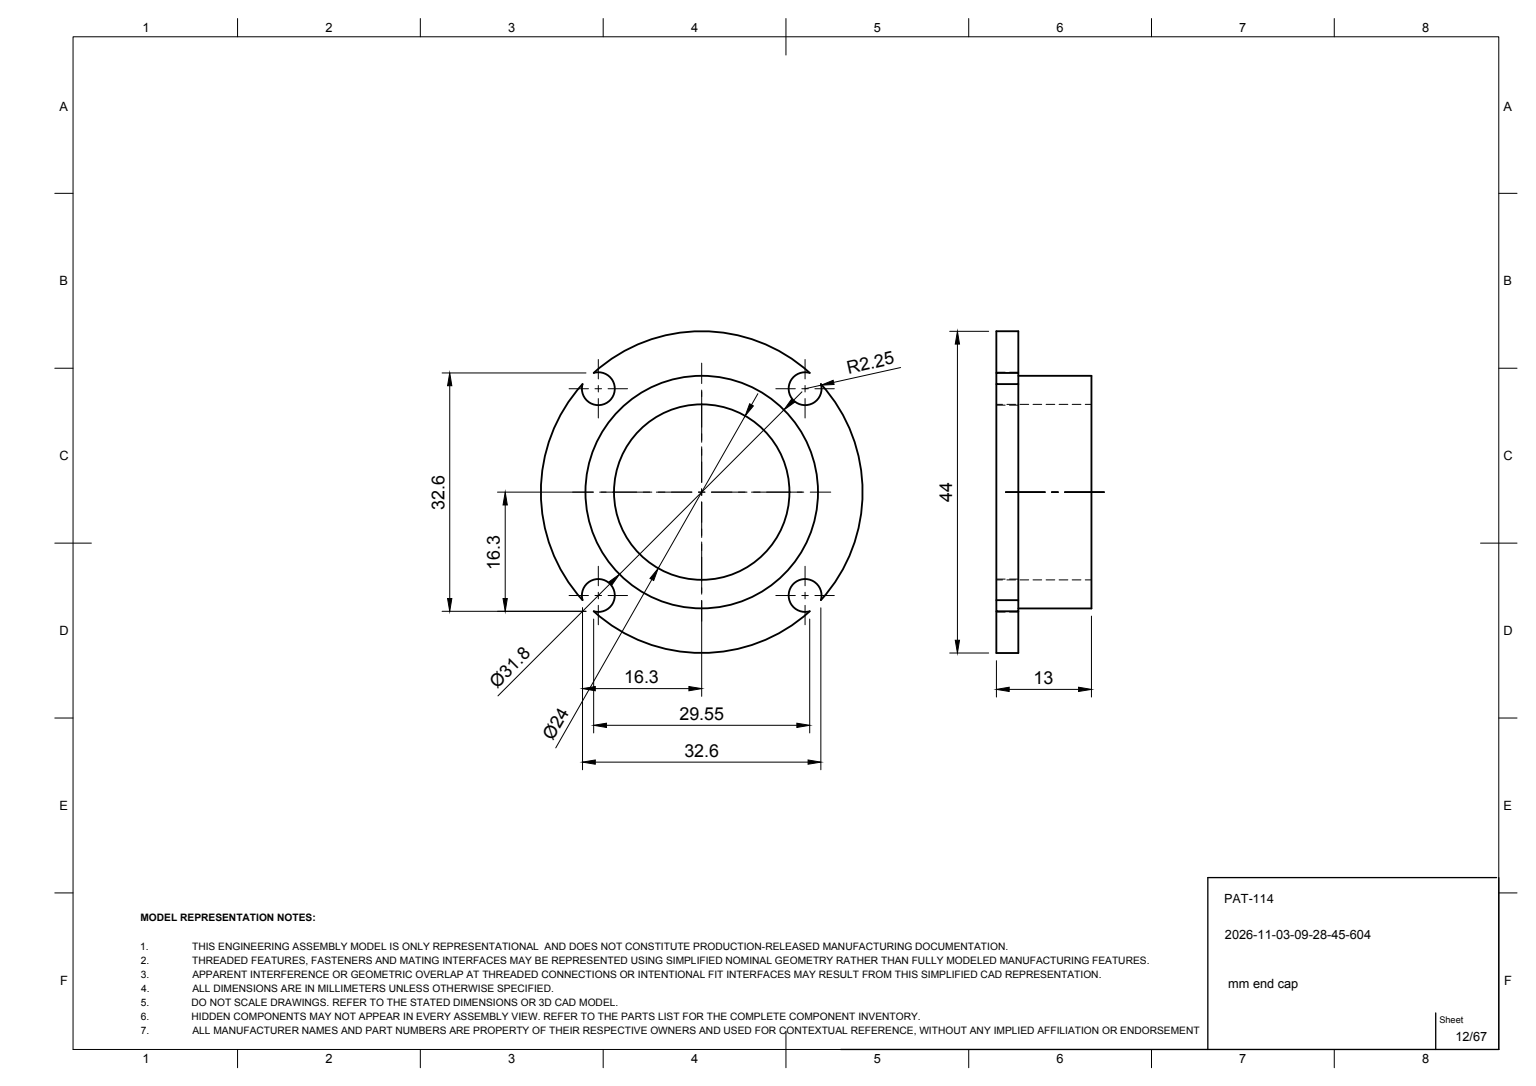
ISO-10303-21;
HEADER;
/* Generated by software containing ST-Developer
 * from STEP Tools, Inc. (www.steptools.com) 
 */

FILE_DESCRIPTION(
/* description */ ('Two-stage gear reducer in split housing'),
/* implementation_level */ '2;1');

FILE_NAME(
/* name */ 'mm end cap.step',
/* time_stamp */ '2026-10-28T03:22:31-07:00',
/* author */ (''),
/* organization */ (''),
/* preprocessor_version */ 'ST-DEVELOPER v20.2',
/* originating_system */ 'Autodesk Translation Framework v15.17.0.0',
/* authorisation */ '');

FILE_SCHEMA (('AUTOMOTIVE_DESIGN { 1 0 10303 214 3 1 1 }'));
ENDSEC;

DATA;
#10=MECHANICAL_DESIGN_GEOMETRIC_PRESENTATION_REPRESENTATION('',(#1241),#73366);
#1129=SHAPE_REPRESENTATION_RELATIONSHIP('SRR','None',#73616,#1185);
#1185=ADVANCED_BREP_SHAPE_REPRESENTATION('',(#1312),#73312);
#1241=STYLED_ITEM('',(#74002),#1312);
#1312=MANIFOLD_SOLID_BREP('Body1',#16129);
#1460=FACE_BOUND('',#3200,.T.);
#1461=FACE_BOUND('',#3207,.T.);
#1462=FACE_BOUND('',#3210,.T.);
#1708=PLANE('',#17204);
#1709=PLANE('',#17221);
#1710=PLANE('',#17224);
#2196=FACE_OUTER_BOUND('',#3195,.T.);
#2197=FACE_OUTER_BOUND('',#3196,.T.);
#2198=FACE_OUTER_BOUND('',#3197,.T.);
#2199=FACE_OUTER_BOUND('',#3198,.T.);
#2200=FACE_OUTER_BOUND('',#3199,.T.);
#2201=FACE_OUTER_BOUND('',#3201,.T.);
#2202=FACE_OUTER_BOUND('',#3202,.T.);
#2203=FACE_OUTER_BOUND('',#3203,.T.);
#2204=FACE_OUTER_BOUND('',#3204,.T.);
#2205=FACE_OUTER_BOUND('',#3205,.T.);
#2206=FACE_OUTER_BOUND('',#3206,.T.);
#2207=FACE_OUTER_BOUND('',#3208,.T.);
#2208=FACE_OUTER_BOUND('',#3209,.T.);
#3195=EDGE_LOOP('',(#11371,#11372,#11373,#11374));
#3196=EDGE_LOOP('',(#11375,#11376,#11377,#11378));
#3197=EDGE_LOOP('',(#11379,#11380,#11381,#11382));
#3198=EDGE_LOOP('',(#11383,#11384,#11385,#11386));
#3199=EDGE_LOOP('',(#11387,#11388,#11389,#11390,#11391,#11392,#11393,#11394));
#3200=EDGE_LOOP('',(#11395));
#3201=EDGE_LOOP('',(#11396,#11397,#11398,#11399));
#3202=EDGE_LOOP('',(#11400,#11401,#11402,#11403));
#3203=EDGE_LOOP('',(#11404,#11405,#11406,#11407));
#3204=EDGE_LOOP('',(#11408,#11409,#11410,#11411));
#3205=EDGE_LOOP('',(#11412,#11413,#11414,#11415));
#3206=EDGE_LOOP('',(#11416));
#3207=EDGE_LOOP('',(#11417));
#3208=EDGE_LOOP('',(#11418,#11419,#11420,#11421));
#3209=EDGE_LOOP('',(#11422,#11423,#11424,#11425,#11426,#11427,#11428,#11429));
#3210=EDGE_LOOP('',(#11430));
#4312=LINE('',#23701,#5336);
#4313=LINE('',#23705,#5337);
#4314=LINE('',#23710,#5338);
#4315=LINE('',#23714,#5339);
#4316=LINE('',#23719,#5340);
#4317=LINE('',#23723,#5341);
#4318=LINE('',#23728,#5342);
#4319=LINE('',#23732,#5343);
#4320=LINE('',#23753,#5344);
#4321=LINE('',#23759,#5345);
#5336=VECTOR('',#19476,1.);
#5337=VECTOR('',#19479,1.);
#5338=VECTOR('',#19484,1.);
#5339=VECTOR('',#19487,1.);
#5340=VECTOR('',#19492,1.);
#5341=VECTOR('',#19495,1.);
#5342=VECTOR('',#19500,1.);
#5343=VECTOR('',#19503,1.);
#5344=VECTOR('',#19538,1.59);
#5345=VECTOR('',#19547,1.2);
#6280=CIRCLE('',#17193,0.225);
#6281=CIRCLE('',#17194,0.225);
#6282=CIRCLE('',#17196,0.225);
#6283=CIRCLE('',#17197,0.225);
#6284=CIRCLE('',#17199,0.225);
#6285=CIRCLE('',#17200,0.225);
#6286=CIRCLE('',#17202,0.225);
#6287=CIRCLE('',#17203,0.225);
#6288=CIRCLE('',#17205,2.2);
#6289=CIRCLE('',#17206,2.2);
#6290=CIRCLE('',#17207,2.2);
#6291=CIRCLE('',#17208,2.2);
#6292=CIRCLE('',#17209,1.2);
#6293=CIRCLE('',#17211,2.2);
#6294=CIRCLE('',#17213,2.2);
#6295=CIRCLE('',#17215,2.2);
#6296=CIRCLE('',#17217,2.2);
#6297=CIRCLE('',#17219,1.59);
#6298=CIRCLE('',#17220,1.59);
#6299=CIRCLE('',#17222,1.2);
#7112=VERTEX_POINT('',#23699);
#7113=VERTEX_POINT('',#23700);
#7114=VERTEX_POINT('',#23702);
#7115=VERTEX_POINT('',#23704);
#7116=VERTEX_POINT('',#23708);
#7117=VERTEX_POINT('',#23709);
#7118=VERTEX_POINT('',#23711);
#7119=VERTEX_POINT('',#23713);
#7120=VERTEX_POINT('',#23717);
#7121=VERTEX_POINT('',#23718);
#7122=VERTEX_POINT('',#23720);
#7123=VERTEX_POINT('',#23722);
#7124=VERTEX_POINT('',#23726);
#7125=VERTEX_POINT('',#23727);
#7126=VERTEX_POINT('',#23729);
#7127=VERTEX_POINT('',#23731);
#7128=VERTEX_POINT('',#23739);
#7129=VERTEX_POINT('',#23750);
#7130=VERTEX_POINT('',#23752);
#7131=VERTEX_POINT('',#23756);
#8739=EDGE_CURVE('',#7112,#7113,#4312,.T.);
#8740=EDGE_CURVE('',#7114,#7112,#6280,.T.);
#8741=EDGE_CURVE('',#7115,#7114,#4313,.T.);
#8742=EDGE_CURVE('',#7113,#7115,#6281,.T.);
#8743=EDGE_CURVE('',#7116,#7117,#4314,.T.);
#8744=EDGE_CURVE('',#7118,#7116,#6282,.T.);
#8745=EDGE_CURVE('',#7119,#7118,#4315,.T.);
#8746=EDGE_CURVE('',#7117,#7119,#6283,.T.);
#8747=EDGE_CURVE('',#7120,#7121,#4316,.T.);
#8748=EDGE_CURVE('',#7122,#7120,#6284,.T.);
#8749=EDGE_CURVE('',#7123,#7122,#4317,.T.);
#8750=EDGE_CURVE('',#7121,#7123,#6285,.T.);
#8751=EDGE_CURVE('',#7124,#7125,#4318,.T.);
#8752=EDGE_CURVE('',#7126,#7124,#6286,.T.);
#8753=EDGE_CURVE('',#7127,#7126,#4319,.T.);
#8754=EDGE_CURVE('',#7125,#7127,#6287,.T.);
#8755=EDGE_CURVE('',#7126,#7112,#6288,.T.);
#8756=EDGE_CURVE('',#7122,#7124,#6289,.T.);
#8757=EDGE_CURVE('',#7118,#7120,#6290,.T.);
#8758=EDGE_CURVE('',#7114,#7116,#6291,.T.);
#8759=EDGE_CURVE('',#7128,#7128,#6292,.T.);
#8760=EDGE_CURVE('',#7123,#7125,#6293,.T.);
#8761=EDGE_CURVE('',#7119,#7121,#6294,.T.);
#8762=EDGE_CURVE('',#7127,#7113,#6295,.T.);
#8763=EDGE_CURVE('',#7115,#7117,#6296,.T.);
#8764=EDGE_CURVE('',#7129,#7129,#6297,.T.);
#8765=EDGE_CURVE('',#7129,#7130,#4320,.T.);
#8766=EDGE_CURVE('',#7130,#7130,#6298,.T.);
#8767=EDGE_CURVE('',#7131,#7131,#6299,.T.);
#8768=EDGE_CURVE('',#7131,#7128,#4321,.T.);
#11371=ORIENTED_EDGE('',*,*,#8739,.F.);
#11372=ORIENTED_EDGE('',*,*,#8740,.F.);
#11373=ORIENTED_EDGE('',*,*,#8741,.F.);
#11374=ORIENTED_EDGE('',*,*,#8742,.F.);
#11375=ORIENTED_EDGE('',*,*,#8743,.F.);
#11376=ORIENTED_EDGE('',*,*,#8744,.F.);
#11377=ORIENTED_EDGE('',*,*,#8745,.F.);
#11378=ORIENTED_EDGE('',*,*,#8746,.F.);
#11379=ORIENTED_EDGE('',*,*,#8747,.F.);
#11380=ORIENTED_EDGE('',*,*,#8748,.F.);
#11381=ORIENTED_EDGE('',*,*,#8749,.F.);
#11382=ORIENTED_EDGE('',*,*,#8750,.F.);
#11383=ORIENTED_EDGE('',*,*,#8751,.F.);
#11384=ORIENTED_EDGE('',*,*,#8752,.F.);
#11385=ORIENTED_EDGE('',*,*,#8753,.F.);
#11386=ORIENTED_EDGE('',*,*,#8754,.F.);
#11387=ORIENTED_EDGE('',*,*,#8740,.T.);
#11388=ORIENTED_EDGE('',*,*,#8755,.F.);
#11389=ORIENTED_EDGE('',*,*,#8752,.T.);
#11390=ORIENTED_EDGE('',*,*,#8756,.F.);
#11391=ORIENTED_EDGE('',*,*,#8748,.T.);
#11392=ORIENTED_EDGE('',*,*,#8757,.F.);
#11393=ORIENTED_EDGE('',*,*,#8744,.T.);
#11394=ORIENTED_EDGE('',*,*,#8758,.F.);
#11395=ORIENTED_EDGE('',*,*,#8759,.F.);
#11396=ORIENTED_EDGE('',*,*,#8749,.T.);
#11397=ORIENTED_EDGE('',*,*,#8756,.T.);
#11398=ORIENTED_EDGE('',*,*,#8751,.T.);
#11399=ORIENTED_EDGE('',*,*,#8760,.F.);
#11400=ORIENTED_EDGE('',*,*,#8745,.T.);
#11401=ORIENTED_EDGE('',*,*,#8757,.T.);
#11402=ORIENTED_EDGE('',*,*,#8747,.T.);
#11403=ORIENTED_EDGE('',*,*,#8761,.F.);
#11404=ORIENTED_EDGE('',*,*,#8739,.T.);
#11405=ORIENTED_EDGE('',*,*,#8762,.F.);
#11406=ORIENTED_EDGE('',*,*,#8753,.T.);
#11407=ORIENTED_EDGE('',*,*,#8755,.T.);
#11408=ORIENTED_EDGE('',*,*,#8741,.T.);
#11409=ORIENTED_EDGE('',*,*,#8758,.T.);
#11410=ORIENTED_EDGE('',*,*,#8743,.T.);
#11411=ORIENTED_EDGE('',*,*,#8763,.F.);
#11412=ORIENTED_EDGE('',*,*,#8764,.F.);
#11413=ORIENTED_EDGE('',*,*,#8765,.T.);
#11414=ORIENTED_EDGE('',*,*,#8766,.F.);
#11415=ORIENTED_EDGE('',*,*,#8765,.F.);
#11416=ORIENTED_EDGE('',*,*,#8764,.T.);
#11417=ORIENTED_EDGE('',*,*,#8767,.T.);
#11418=ORIENTED_EDGE('',*,*,#8767,.F.);
#11419=ORIENTED_EDGE('',*,*,#8768,.T.);
#11420=ORIENTED_EDGE('',*,*,#8759,.T.);
#11421=ORIENTED_EDGE('',*,*,#8768,.F.);
#11422=ORIENTED_EDGE('',*,*,#8742,.T.);
#11423=ORIENTED_EDGE('',*,*,#8763,.T.);
#11424=ORIENTED_EDGE('',*,*,#8746,.T.);
#11425=ORIENTED_EDGE('',*,*,#8761,.T.);
#11426=ORIENTED_EDGE('',*,*,#8750,.T.);
#11427=ORIENTED_EDGE('',*,*,#8760,.T.);
#11428=ORIENTED_EDGE('',*,*,#8754,.T.);
#11429=ORIENTED_EDGE('',*,*,#8762,.T.);
#11430=ORIENTED_EDGE('',*,*,#8766,.T.);
#14995=CYLINDRICAL_SURFACE('',#17192,0.225);
#14996=CYLINDRICAL_SURFACE('',#17195,0.225);
#14997=CYLINDRICAL_SURFACE('',#17198,0.225);
#14998=CYLINDRICAL_SURFACE('',#17201,0.225);
#14999=CYLINDRICAL_SURFACE('',#17210,2.2);
#15000=CYLINDRICAL_SURFACE('',#17212,2.2);
#15001=CYLINDRICAL_SURFACE('',#17214,2.2);
#15002=CYLINDRICAL_SURFACE('',#17216,2.2);
#15003=CYLINDRICAL_SURFACE('',#17218,1.59);
#15004=CYLINDRICAL_SURFACE('',#17223,1.2);
#15403=ADVANCED_FACE('',(#2196),#14995,.F.);
#15404=ADVANCED_FACE('',(#2197),#14996,.F.);
#15405=ADVANCED_FACE('',(#2198),#14997,.F.);
#15406=ADVANCED_FACE('',(#2199),#14998,.F.);
#15407=ADVANCED_FACE('',(#2200,#1460),#1708,.F.);
#15408=ADVANCED_FACE('',(#2201),#14999,.T.);
#15409=ADVANCED_FACE('',(#2202),#15000,.T.);
#15410=ADVANCED_FACE('',(#2203),#15001,.T.);
#15411=ADVANCED_FACE('',(#2204),#15002,.T.);
#15412=ADVANCED_FACE('',(#2205),#15003,.T.);
#15413=ADVANCED_FACE('',(#2206,#1461),#1709,.T.);
#15414=ADVANCED_FACE('',(#2207),#15004,.F.);
#15415=ADVANCED_FACE('',(#2208,#1462),#1710,.T.);
#16129=CLOSED_SHELL('',(#15403,#15404,#15405,#15406,#15407,#15408,#15409,
#15410,#15411,#15412,#15413,#15414,#15415));
#17191=AXIS2_PLACEMENT_3D('',#23697,#19472,#19473);
#17192=AXIS2_PLACEMENT_3D('',#23698,#19474,#19475);
#17193=AXIS2_PLACEMENT_3D('',#23703,#19477,#19478);
#17194=AXIS2_PLACEMENT_3D('',#23706,#19480,#19481);
#17195=AXIS2_PLACEMENT_3D('',#23707,#19482,#19483);
#17196=AXIS2_PLACEMENT_3D('',#23712,#19485,#19486);
#17197=AXIS2_PLACEMENT_3D('',#23715,#19488,#19489);
#17198=AXIS2_PLACEMENT_3D('',#23716,#19490,#19491);
#17199=AXIS2_PLACEMENT_3D('',#23721,#19493,#19494);
#17200=AXIS2_PLACEMENT_3D('',#23724,#19496,#19497);
#17201=AXIS2_PLACEMENT_3D('',#23725,#19498,#19499);
#17202=AXIS2_PLACEMENT_3D('',#23730,#19501,#19502);
#17203=AXIS2_PLACEMENT_3D('',#23733,#19504,#19505);
#17204=AXIS2_PLACEMENT_3D('',#23734,#19506,#19507);
#17205=AXIS2_PLACEMENT_3D('',#23735,#19508,#19509);
#17206=AXIS2_PLACEMENT_3D('',#23736,#19510,#19511);
#17207=AXIS2_PLACEMENT_3D('',#23737,#19512,#19513);
#17208=AXIS2_PLACEMENT_3D('',#23738,#19514,#19515);
#17209=AXIS2_PLACEMENT_3D('',#23740,#19516,#19517);
#17210=AXIS2_PLACEMENT_3D('',#23741,#19518,#19519);
#17211=AXIS2_PLACEMENT_3D('',#23742,#19520,#19521);
#17212=AXIS2_PLACEMENT_3D('',#23743,#19522,#19523);
#17213=AXIS2_PLACEMENT_3D('',#23744,#19524,#19525);
#17214=AXIS2_PLACEMENT_3D('',#23745,#19526,#19527);
#17215=AXIS2_PLACEMENT_3D('',#23746,#19528,#19529);
#17216=AXIS2_PLACEMENT_3D('',#23747,#19530,#19531);
#17217=AXIS2_PLACEMENT_3D('',#23748,#19532,#19533);
#17218=AXIS2_PLACEMENT_3D('',#23749,#19534,#19535);
#17219=AXIS2_PLACEMENT_3D('',#23751,#19536,#19537);
#17220=AXIS2_PLACEMENT_3D('',#23754,#19539,#19540);
#17221=AXIS2_PLACEMENT_3D('',#23755,#19541,#19542);
#17222=AXIS2_PLACEMENT_3D('',#23757,#19543,#19544);
#17223=AXIS2_PLACEMENT_3D('',#23758,#19545,#19546);
#17224=AXIS2_PLACEMENT_3D('',#23760,#19548,#19549);
#19472=DIRECTION('axis',(0.,0.,1.));
#19473=DIRECTION('refdir',(1.,0.,0.));
#19474=DIRECTION('center_axis',(0.,1.,0.));
#19475=DIRECTION('ref_axis',(0.707106781186543,0.,0.707106781186552));
#19476=DIRECTION('',(0.,1.,0.));
#19477=DIRECTION('center_axis',(0.,1.,0.));
#19478=DIRECTION('ref_axis',(1.,0.,0.));
#19479=DIRECTION('',(0.,-1.,0.));
#19480=DIRECTION('center_axis',(0.,-1.,0.));
#19481=DIRECTION('ref_axis',(1.,0.,0.));
#19482=DIRECTION('center_axis',(0.,1.,0.));
#19483=DIRECTION('ref_axis',(0.707106781186542,0.,-0.707106781186553));
#19484=DIRECTION('',(0.,1.,0.));
#19485=DIRECTION('center_axis',(0.,1.,0.));
#19486=DIRECTION('ref_axis',(1.,0.,0.));
#19487=DIRECTION('',(0.,-1.,0.));
#19488=DIRECTION('center_axis',(0.,-1.,0.));
#19489=DIRECTION('ref_axis',(1.,0.,0.));
#19490=DIRECTION('center_axis',(0.,1.,0.));
#19491=DIRECTION('ref_axis',(-0.707106781186542,0.,-0.707106781186553));
#19492=DIRECTION('',(0.,1.,0.));
#19493=DIRECTION('center_axis',(0.,1.,0.));
#19494=DIRECTION('ref_axis',(1.,0.,0.));
#19495=DIRECTION('',(0.,-1.,0.));
#19496=DIRECTION('center_axis',(0.,-1.,0.));
#19497=DIRECTION('ref_axis',(1.,0.,0.));
#19498=DIRECTION('center_axis',(0.,1.,0.));
#19499=DIRECTION('ref_axis',(-0.707106781186549,0.,0.707106781186546));
#19500=DIRECTION('',(0.,1.,0.));
#19501=DIRECTION('center_axis',(0.,1.,0.));
#19502=DIRECTION('ref_axis',(1.,0.,0.));
#19503=DIRECTION('',(0.,-1.,0.));
#19504=DIRECTION('center_axis',(0.,-1.,0.));
#19505=DIRECTION('ref_axis',(1.,0.,0.));
#19506=DIRECTION('center_axis',(0.,1.,0.));
#19507=DIRECTION('ref_axis',(1.,0.,0.));
#19508=DIRECTION('center_axis',(0.,1.,0.));
#19509=DIRECTION('ref_axis',(1.,0.,0.));
#19510=DIRECTION('center_axis',(0.,1.,0.));
#19511=DIRECTION('ref_axis',(1.,0.,0.));
#19512=DIRECTION('center_axis',(0.,1.,0.));
#19513=DIRECTION('ref_axis',(1.,0.,0.));
#19514=DIRECTION('center_axis',(0.,1.,0.));
#19515=DIRECTION('ref_axis',(1.,0.,0.));
#19516=DIRECTION('center_axis',(0.,-1.,0.));
#19517=DIRECTION('ref_axis',(1.,0.,0.));
#19518=DIRECTION('center_axis',(0.,1.,0.));
#19519=DIRECTION('ref_axis',(1.,0.,0.));
#19520=DIRECTION('center_axis',(0.,1.,0.));
#19521=DIRECTION('ref_axis',(1.,0.,0.));
#19522=DIRECTION('center_axis',(0.,1.,0.));
#19523=DIRECTION('ref_axis',(1.,0.,0.));
#19524=DIRECTION('center_axis',(0.,1.,0.));
#19525=DIRECTION('ref_axis',(1.,0.,0.));
#19526=DIRECTION('center_axis',(0.,1.,0.));
#19527=DIRECTION('ref_axis',(1.,0.,0.));
#19528=DIRECTION('center_axis',(0.,1.,0.));
#19529=DIRECTION('ref_axis',(1.,0.,0.));
#19530=DIRECTION('center_axis',(0.,1.,0.));
#19531=DIRECTION('ref_axis',(-1.,0.,3.21624529935327E-16));
#19532=DIRECTION('center_axis',(0.,1.,0.));
#19533=DIRECTION('ref_axis',(1.,0.,0.));
#19534=DIRECTION('center_axis',(0.,1.,0.));
#19535=DIRECTION('ref_axis',(1.,0.,0.));
#19536=DIRECTION('center_axis',(0.,1.,0.));
#19537=DIRECTION('ref_axis',(1.,0.,0.));
#19538=DIRECTION('',(0.,-1.,0.));
#19539=DIRECTION('center_axis',(0.,-1.,0.));
#19540=DIRECTION('ref_axis',(1.,0.,0.));
#19541=DIRECTION('center_axis',(0.,1.,0.));
#19542=DIRECTION('ref_axis',(1.,0.,0.));
#19543=DIRECTION('center_axis',(0.,-1.,0.));
#19544=DIRECTION('ref_axis',(1.,0.,0.));
#19545=DIRECTION('center_axis',(0.,1.,0.));
#19546=DIRECTION('ref_axis',(1.,0.,0.));
#19547=DIRECTION('',(0.,-1.,0.));
#19548=DIRECTION('center_axis',(0.,1.,0.));
#19549=DIRECTION('ref_axis',(1.,0.,0.));
#23697=CARTESIAN_POINT('',(0.,0.,0.));
#23698=CARTESIAN_POINT('Origin',(-1.4142135623731,-7.9,8.5857864376269));
#23699=CARTESIAN_POINT('',(-1.47733531993816,-7.8,8.3698219874924));
#23700=CARTESIAN_POINT('',(-1.47733531993816,-7.5,8.3698219874924));
#23701=CARTESIAN_POINT('',(-1.47733531993816,-7.9,8.3698219874924));
#23702=CARTESIAN_POINT('',(-1.6301780125076,-7.8,8.52266468006184));
#23703=CARTESIAN_POINT('Origin',(-1.4142135623731,-7.8,8.5857864376269));
#23704=CARTESIAN_POINT('',(-1.6301780125076,-7.5,8.52266468006184));
#23705=CARTESIAN_POINT('',(-1.6301780125076,-7.9,8.52266468006184));
#23706=CARTESIAN_POINT('Origin',(-1.4142135623731,-7.5,8.5857864376269));
#23707=CARTESIAN_POINT('Origin',(-1.41421356237309,-7.9,11.4142135623731));
#23708=CARTESIAN_POINT('',(-1.6301780125076,-7.8,11.4773353199382));
#23709=CARTESIAN_POINT('',(-1.6301780125076,-7.5,11.4773353199382));
#23710=CARTESIAN_POINT('',(-1.6301780125076,-7.9,11.4773353199382));
#23711=CARTESIAN_POINT('',(-1.47733531993816,-7.8,11.6301780125076));
#23712=CARTESIAN_POINT('Origin',(-1.41421356237309,-7.8,11.4142135623731));
#23713=CARTESIAN_POINT('',(-1.47733531993816,-7.5,11.6301780125076));
#23714=CARTESIAN_POINT('',(-1.47733531993816,-7.9,11.6301780125076));
#23715=CARTESIAN_POINT('Origin',(-1.41421356237309,-7.5,11.4142135623731));
#23716=CARTESIAN_POINT('Origin',(1.4142135623731,-7.9,11.4142135623731));
#23717=CARTESIAN_POINT('',(1.47733531993816,-7.8,11.6301780125076));
#23718=CARTESIAN_POINT('',(1.47733531993816,-7.5,11.6301780125076));
#23719=CARTESIAN_POINT('',(1.47733531993816,-7.9,11.6301780125076));
#23720=CARTESIAN_POINT('',(1.6301780125076,-7.8,11.4773353199382));
#23721=CARTESIAN_POINT('Origin',(1.4142135623731,-7.8,11.4142135623731));
#23722=CARTESIAN_POINT('',(1.6301780125076,-7.5,11.4773353199382));
#23723=CARTESIAN_POINT('',(1.6301780125076,-7.9,11.4773353199382));
#23724=CARTESIAN_POINT('Origin',(1.4142135623731,-7.5,11.4142135623731));
#23725=CARTESIAN_POINT('Origin',(1.41421356237309,-7.9,8.5857864376269));
#23726=CARTESIAN_POINT('',(1.6301780125076,-7.8,8.52266468006184));
#23727=CARTESIAN_POINT('',(1.6301780125076,-7.5,8.52266468006184));
#23728=CARTESIAN_POINT('',(1.6301780125076,-7.9,8.52266468006184));
#23729=CARTESIAN_POINT('',(1.47733531993816,-7.8,8.3698219874924));
#23730=CARTESIAN_POINT('Origin',(1.41421356237309,-7.8,8.5857864376269));
#23731=CARTESIAN_POINT('',(1.47733531993816,-7.5,8.3698219874924));
#23732=CARTESIAN_POINT('',(1.47733531993816,-7.9,8.3698219874924));
#23733=CARTESIAN_POINT('Origin',(1.41421356237309,-7.5,8.5857864376269));
#23734=CARTESIAN_POINT('Origin',(0.,-7.8,10.));
#23735=CARTESIAN_POINT('Origin',(0.,-7.8,10.));
#23736=CARTESIAN_POINT('Origin',(0.,-7.8,10.));
#23737=CARTESIAN_POINT('Origin',(0.,-7.8,10.));
#23738=CARTESIAN_POINT('Origin',(0.,-7.8,10.));
#23739=CARTESIAN_POINT('',(-1.2,-7.8,10.));
#23740=CARTESIAN_POINT('Origin',(0.,-7.8,10.));
#23741=CARTESIAN_POINT('Origin',(0.,-7.8,10.));
#23742=CARTESIAN_POINT('Origin',(0.,-7.5,10.));
#23743=CARTESIAN_POINT('Origin',(0.,-7.8,10.));
#23744=CARTESIAN_POINT('Origin',(0.,-7.5,10.));
#23745=CARTESIAN_POINT('Origin',(0.,-7.8,10.));
#23746=CARTESIAN_POINT('Origin',(0.,-7.5,10.));
#23747=CARTESIAN_POINT('Origin',(0.,-7.8,10.));
#23748=CARTESIAN_POINT('Origin',(0.,-7.5,10.));
#23749=CARTESIAN_POINT('Origin',(0.,-7.5,10.));
#23750=CARTESIAN_POINT('',(-1.59,-6.5,10.));
#23751=CARTESIAN_POINT('Origin',(0.,-6.5,10.));
#23752=CARTESIAN_POINT('',(-1.59,-7.5,10.));
#23753=CARTESIAN_POINT('',(-1.59,-7.5,10.));
#23754=CARTESIAN_POINT('Origin',(0.,-7.5,10.));
#23755=CARTESIAN_POINT('Origin',(0.,-6.5,10.));
#23756=CARTESIAN_POINT('',(-1.2,-6.5,10.));
#23757=CARTESIAN_POINT('Origin',(0.,-6.5,10.));
#23758=CARTESIAN_POINT('Origin',(0.,-7.8,10.));
#23759=CARTESIAN_POINT('',(-1.2,-7.8,10.));
#23760=CARTESIAN_POINT('Origin',(0.,-7.5,10.));
#73248=UNCERTAINTY_MEASURE_WITH_UNIT(LENGTH_MEASURE(0.001),#73367,
'DISTANCE_ACCURACY_VALUE',
'Maximum model space distance between geometric entities at asserted c
onnectivities');
#73302=UNCERTAINTY_MEASURE_WITH_UNIT(LENGTH_MEASURE(0.001),#73367,
'DISTANCE_ACCURACY_VALUE',
'Maximum model space distance between geometric entities at asserted c
onnectivities');
#73312=(
GEOMETRIC_REPRESENTATION_CONTEXT(3)
GLOBAL_UNCERTAINTY_ASSIGNED_CONTEXT((#73248))
GLOBAL_UNIT_ASSIGNED_CONTEXT((#73367,#73369,#73370))
REPRESENTATION_CONTEXT('','3D')
);
#73366=(
GEOMETRIC_REPRESENTATION_CONTEXT(3)
GLOBAL_UNCERTAINTY_ASSIGNED_CONTEXT((#73302))
GLOBAL_UNIT_ASSIGNED_CONTEXT((#73367,#73369,#73370))
REPRESENTATION_CONTEXT('','3D')
);
#73367=(
LENGTH_UNIT()
NAMED_UNIT(*)
SI_UNIT(.CENTI.,.METRE.)
);
#73369=(
NAMED_UNIT(*)
PLANE_ANGLE_UNIT()
SI_UNIT($,.RADIAN.)
);
#73370=(
NAMED_UNIT(*)
SI_UNIT($,.STERADIAN.)
SOLID_ANGLE_UNIT()
);
#73380=SHAPE_DEFINITION_REPRESENTATION(#73443,#73616);
#73443=PRODUCT_DEFINITION_SHAPE('',$,#73680);
#73616=SHAPE_REPRESENTATION('',(#17191),#73312);
#73670=PRODUCT_DEFINITION_CONTEXT('part definition',#73861,'design');
#73680=PRODUCT_DEFINITION('mm end cap','mm end cap',#73743,#73670);
#73743=PRODUCT_DEFINITION_FORMATION('',$,#73872);
#73861=APPLICATION_CONTEXT(
'Core Data for Automotive Mechanical Design Process');
#73862=PRODUCT_CONTEXT('part definition',#73861,'mechanical');
#73872=PRODUCT('mm end cap','mm end cap','mm end cap',(#73862));
#73996=COLOUR_RGB('Off White',0.89,0.88,0.83);
#73997=FILL_AREA_STYLE_COLOUR('',#73996);
#73998=FILL_AREA_STYLE('',(#73997));
#73999=SURFACE_STYLE_FILL_AREA(#73998);
#74000=SURFACE_SIDE_STYLE('',(#73999));
#74001=SURFACE_STYLE_USAGE(.BOTH.,#74000);
#74002=PRESENTATION_STYLE_ASSIGNMENT((#74001));
ENDSEC;
END-ISO-10303-21;
